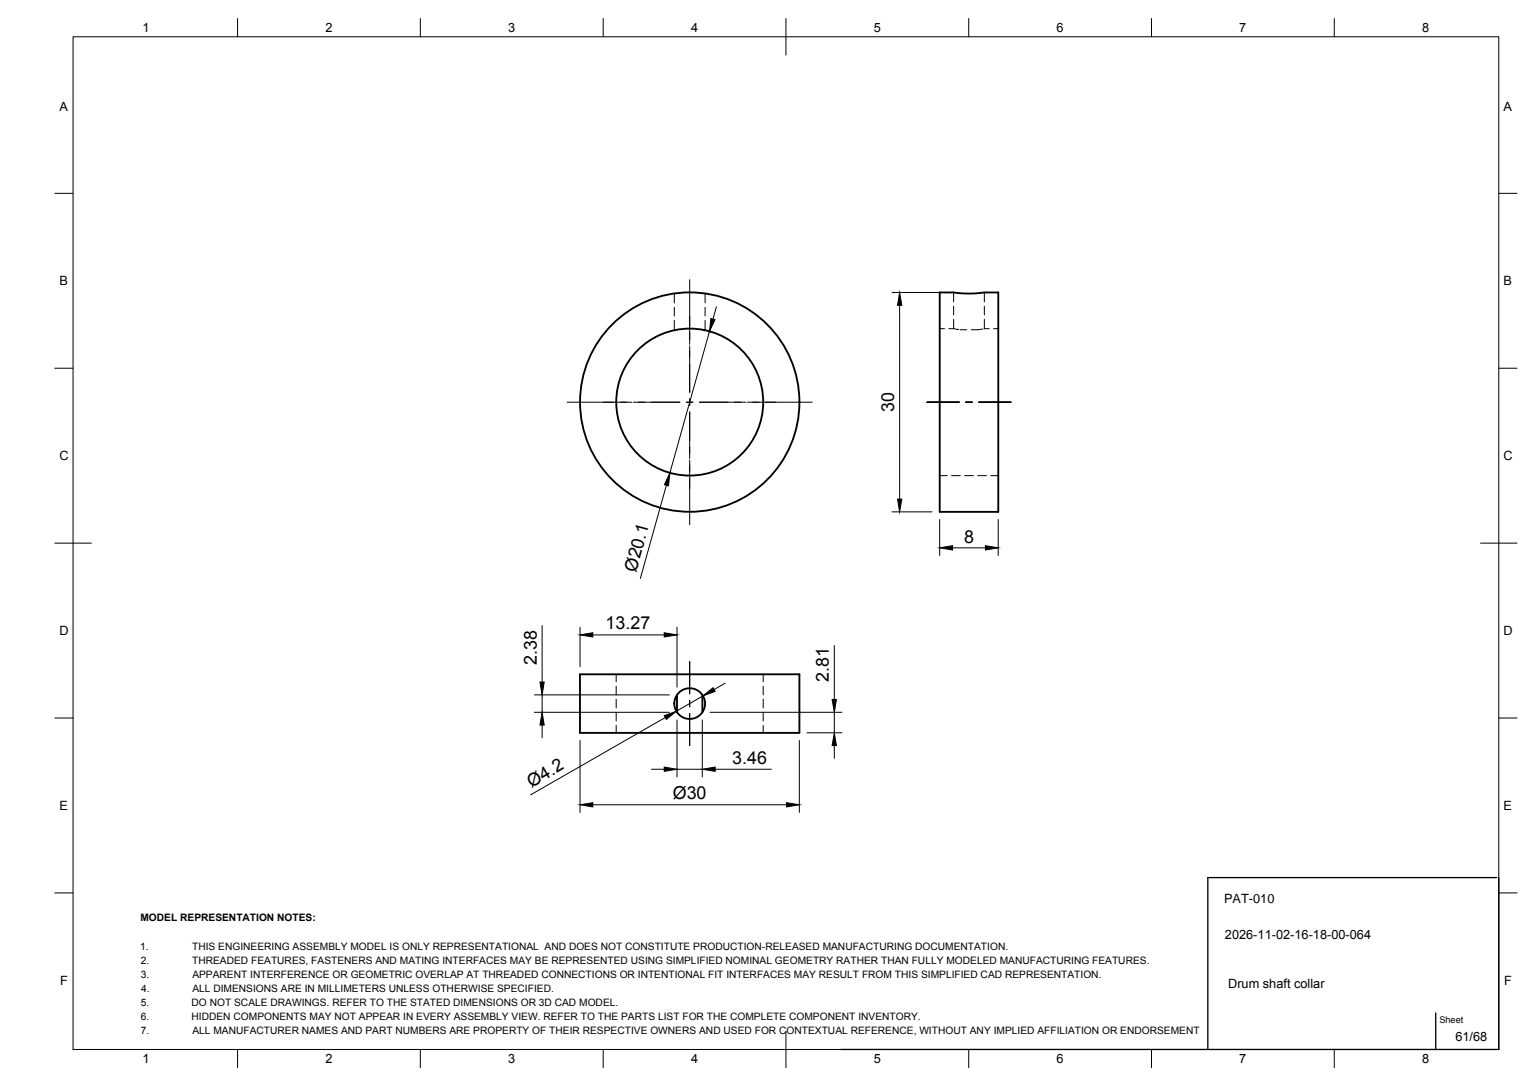
ISO-10303-21;
HEADER;
/* Generated by software containing ST-Developer
 * from STEP Tools, Inc. (www.steptools.com) 
 */

FILE_DESCRIPTION(
/* description */ ('Belt conveyor head drive unit'),
/* implementation_level */ '2;1');

FILE_NAME(
/* name */ 'Drum shaft collar.step',
/* time_stamp */ '2026-10-28T03:26:19-07:00',
/* author */ (''),
/* organization */ (''),
/* preprocessor_version */ 'ST-DEVELOPER v20.2',
/* originating_system */ 'Autodesk Translation Framework v15.17.0.0',
/* authorisation */ '');

FILE_SCHEMA (('AUTOMOTIVE_DESIGN { 1 0 10303 214 3 1 1 }'));
ENDSEC;

DATA;
#10=MECHANICAL_DESIGN_GEOMETRIC_PRESENTATION_REPRESENTATION('',(#922),#27069);
#607=B_SPLINE_CURVE_WITH_KNOTS('',3,(#25420,#25421,#25422,#25423,#25424,
#25425,#25426,#25427,#25428,#25429,#25430,#25431,#25432,#25433),
 .UNSPECIFIED.,.F.,.F.,(4,2,2,2,2,2,4),(0.756005737987021,0.793568827564646,
0.872922520054201,0.952276212543756,1.03162990503331,1.11098359752286,1.14854668710049),
 .UNSPECIFIED.);
#608=B_SPLINE_CURVE_WITH_KNOTS('',3,(#25439,#25440,#25441,#25442,#25443,
#25444,#25445,#25446,#25447,#25448,#25449,#25450,#25451,#25452,#25453,#25454,
#25455,#25456),.UNSPECIFIED.,.F.,.F.,(4,2,2,2,2,2,2,2,4),(0.,0.0792165807733631,
0.158433161546726,0.23764869707457,0.316864232602414,0.396079768130258,
0.475295303658102,0.554511884431466,0.633728465204829),.UNSPECIFIED.);
#609=B_SPLINE_CURVE_WITH_KNOTS('',3,(#25457,#25458,#25459,#25460,#25461,
#25462,#25463,#25464,#25465,#25466,#25467,#25468,#25469,#25470,#25471,#25472,
#25473,#25474),.UNSPECIFIED.,.F.,.F.,(4,2,2,2,2,2,2,2,4),(0.633728465204829,
0.712945045978192,0.792161626751554,0.871377162279399,0.950592697807243,
1.02980823333509,1.10902376886293,1.18824034963629,1.26745693040966),
 .UNSPECIFIED.);
#610=B_SPLINE_CURVE_WITH_KNOTS('',3,(#25477,#25478,#25479,#25480,#25481,
#25482,#25483,#25484,#25485,#25486,#25487,#25488,#25489,#25490),
 .UNSPECIFIED.,.F.,.F.,(4,2,2,2,2,2,4),(0.121154929624517,0.158718019202143,
0.238071711691697,0.317425404181252,0.396779096670806,0.476132789160361,
0.513695878737986),.UNSPECIFIED.);
#768=SHAPE_REPRESENTATION_RELATIONSHIP('SRR','None',#27417,#837);
#837=ADVANCED_BREP_SHAPE_REPRESENTATION('',(#1003),#27059);
#922=STYLED_ITEM('',(#27797),#1003);
#1003=MANIFOLD_SOLID_BREP('Body1',#13791);
#1242=FACE_BOUND('',#3305,.T.);
#1243=FACE_BOUND('',#3307,.T.);
#1244=FACE_BOUND('',#3309,.T.);
#1245=FACE_BOUND('',#3311,.T.);
#1586=PLANE('',#15930);
#1587=PLANE('',#15935);
#1588=PLANE('',#15942);
#1589=PLANE('',#15943);
#2271=FACE_OUTER_BOUND('',#3301,.T.);
#2272=FACE_OUTER_BOUND('',#3302,.T.);
#2273=FACE_OUTER_BOUND('',#3303,.T.);
#2274=FACE_OUTER_BOUND('',#3304,.T.);
#2275=FACE_OUTER_BOUND('',#3306,.T.);
#2276=FACE_OUTER_BOUND('',#3308,.T.);
#2277=FACE_OUTER_BOUND('',#3310,.T.);
#3301=EDGE_LOOP('',(#11694,#11695));
#3302=EDGE_LOOP('',(#11696,#11697,#11698,#11699,#11700,#11701,#11702,#11703,
#11704));
#3303=EDGE_LOOP('',(#11705,#11706,#11707));
#3304=EDGE_LOOP('',(#11708,#11709,#11710,#11711));
#3305=EDGE_LOOP('',(#11712,#11713,#11714,#11715));
#3306=EDGE_LOOP('',(#11716,#11717,#11718,#11719));
#3307=EDGE_LOOP('',(#11720,#11721));
#3308=EDGE_LOOP('',(#11722));
#3309=EDGE_LOOP('',(#11723));
#3310=EDGE_LOOP('',(#11724));
#3311=EDGE_LOOP('',(#11725));
#4129=LINE('',#25416,#4921);
#4130=LINE('',#25437,#4922);
#4131=LINE('',#25492,#4923);
#4132=LINE('',#25497,#4924);
#4133=LINE('',#25503,#4925);
#4921=VECTOR('',#19803,1.);
#4922=VECTOR('',#19810,0.21);
#4923=VECTOR('',#19815,1.);
#4924=VECTOR('',#19820,1.005);
#4925=VECTOR('',#19827,1.5);
#5733=CIRCLE('',#15931,0.21);
#5734=CIRCLE('',#15933,0.21);
#5735=CIRCLE('',#15934,0.21);
#5736=CIRCLE('',#15937,1.005);
#5737=CIRCLE('',#15938,1.005);
#5738=CIRCLE('',#15940,1.5);
#5739=CIRCLE('',#15941,1.5);
#6889=VERTEX_POINT('',#25414);
#6890=VERTEX_POINT('',#25415);
#6891=VERTEX_POINT('',#25419);
#6892=VERTEX_POINT('',#25434);
#6893=VERTEX_POINT('',#25436);
#6894=VERTEX_POINT('',#25438);
#6895=VERTEX_POINT('',#25475);
#6896=VERTEX_POINT('',#25494);
#6897=VERTEX_POINT('',#25496);
#6898=VERTEX_POINT('',#25500);
#6899=VERTEX_POINT('',#25502);
#8539=EDGE_CURVE('',#6889,#6890,#4129,.T.);
#8540=EDGE_CURVE('',#6889,#6890,#5733,.T.);
#8541=EDGE_CURVE('',#6891,#6889,#607,.T.);
#8542=EDGE_CURVE('',#6892,#6891,#5734,.T.);
#8543=EDGE_CURVE('',#6892,#6893,#4130,.T.);
#8544=EDGE_CURVE('',#6894,#6893,#608,.T.);
#8545=EDGE_CURVE('',#6893,#6894,#609,.T.);
#8546=EDGE_CURVE('',#6895,#6892,#5735,.T.);
#8547=EDGE_CURVE('',#6890,#6895,#610,.T.);
#8548=EDGE_CURVE('',#6895,#6891,#4131,.T.);
#8549=EDGE_CURVE('',#6896,#6896,#5736,.T.);
#8550=EDGE_CURVE('',#6896,#6897,#4132,.T.);
#8551=EDGE_CURVE('',#6897,#6897,#5737,.T.);
#8552=EDGE_CURVE('',#6898,#6898,#5738,.T.);
#8553=EDGE_CURVE('',#6898,#6899,#4133,.T.);
#8554=EDGE_CURVE('',#6899,#6899,#5739,.T.);
#11694=ORIENTED_EDGE('',*,*,#8539,.F.);
#11695=ORIENTED_EDGE('',*,*,#8540,.T.);
#11696=ORIENTED_EDGE('',*,*,#8541,.F.);
#11697=ORIENTED_EDGE('',*,*,#8542,.F.);
#11698=ORIENTED_EDGE('',*,*,#8543,.T.);
#11699=ORIENTED_EDGE('',*,*,#8544,.F.);
#11700=ORIENTED_EDGE('',*,*,#8545,.F.);
#11701=ORIENTED_EDGE('',*,*,#8543,.F.);
#11702=ORIENTED_EDGE('',*,*,#8546,.F.);
#11703=ORIENTED_EDGE('',*,*,#8547,.F.);
#11704=ORIENTED_EDGE('',*,*,#8540,.F.);
#11705=ORIENTED_EDGE('',*,*,#8548,.F.);
#11706=ORIENTED_EDGE('',*,*,#8546,.T.);
#11707=ORIENTED_EDGE('',*,*,#8542,.T.);
#11708=ORIENTED_EDGE('',*,*,#8549,.F.);
#11709=ORIENTED_EDGE('',*,*,#8550,.T.);
#11710=ORIENTED_EDGE('',*,*,#8551,.T.);
#11711=ORIENTED_EDGE('',*,*,#8550,.F.);
#11712=ORIENTED_EDGE('',*,*,#8547,.T.);
#11713=ORIENTED_EDGE('',*,*,#8548,.T.);
#11714=ORIENTED_EDGE('',*,*,#8541,.T.);
#11715=ORIENTED_EDGE('',*,*,#8539,.T.);
#11716=ORIENTED_EDGE('',*,*,#8552,.F.);
#11717=ORIENTED_EDGE('',*,*,#8553,.T.);
#11718=ORIENTED_EDGE('',*,*,#8554,.T.);
#11719=ORIENTED_EDGE('',*,*,#8553,.F.);
#11720=ORIENTED_EDGE('',*,*,#8544,.T.);
#11721=ORIENTED_EDGE('',*,*,#8545,.T.);
#11722=ORIENTED_EDGE('',*,*,#8552,.T.);
#11723=ORIENTED_EDGE('',*,*,#8549,.T.);
#11724=ORIENTED_EDGE('',*,*,#8554,.F.);
#11725=ORIENTED_EDGE('',*,*,#8551,.F.);
#12803=CYLINDRICAL_SURFACE('',#15932,0.21);
#12804=CYLINDRICAL_SURFACE('',#15936,1.005);
#12805=CYLINDRICAL_SURFACE('',#15939,1.5);
#13550=ADVANCED_FACE('',(#2271),#1586,.T.);
#13551=ADVANCED_FACE('',(#2272),#12803,.F.);
#13552=ADVANCED_FACE('',(#2273),#1587,.T.);
#13553=ADVANCED_FACE('',(#2274,#1242),#12804,.F.);
#13554=ADVANCED_FACE('',(#2275,#1243),#12805,.T.);
#13555=ADVANCED_FACE('',(#2276,#1244),#1588,.T.);
#13556=ADVANCED_FACE('',(#2277,#1245),#1589,.F.);
#13791=CLOSED_SHELL('',(#13550,#13551,#13552,#13553,#13554,#13555,#13556));
#15929=AXIS2_PLACEMENT_3D('',#25412,#19799,#19800);
#15930=AXIS2_PLACEMENT_3D('',#25413,#19801,#19802);
#15931=AXIS2_PLACEMENT_3D('',#25417,#19804,#19805);
#15932=AXIS2_PLACEMENT_3D('',#25418,#19806,#19807);
#15933=AXIS2_PLACEMENT_3D('',#25435,#19808,#19809);
#15934=AXIS2_PLACEMENT_3D('',#25476,#19811,#19812);
#15935=AXIS2_PLACEMENT_3D('',#25491,#19813,#19814);
#15936=AXIS2_PLACEMENT_3D('',#25493,#19816,#19817);
#15937=AXIS2_PLACEMENT_3D('',#25495,#19818,#19819);
#15938=AXIS2_PLACEMENT_3D('',#25498,#19821,#19822);
#15939=AXIS2_PLACEMENT_3D('',#25499,#19823,#19824);
#15940=AXIS2_PLACEMENT_3D('',#25501,#19825,#19826);
#15941=AXIS2_PLACEMENT_3D('',#25504,#19828,#19829);
#15942=AXIS2_PLACEMENT_3D('',#25505,#19830,#19831);
#15943=AXIS2_PLACEMENT_3D('',#25506,#19832,#19833);
#19799=DIRECTION('axis',(0.,0.,1.));
#19800=DIRECTION('refdir',(1.,0.,0.));
#19801=DIRECTION('center_axis',(0.,0.,1.));
#19802=DIRECTION('ref_axis',(1.,0.,0.));
#19803=DIRECTION('',(0.,1.,0.));
#19804=DIRECTION('center_axis',(0.,0.,1.));
#19805=DIRECTION('ref_axis',(1.,0.,0.));
#19806=DIRECTION('center_axis',(0.,0.,1.));
#19807=DIRECTION('ref_axis',(1.,0.,0.));
#19808=DIRECTION('center_axis',(0.,0.,1.));
#19809=DIRECTION('ref_axis',(1.,0.,0.));
#19810=DIRECTION('',(0.,0.,1.));
#19811=DIRECTION('center_axis',(0.,0.,1.));
#19812=DIRECTION('ref_axis',(1.,0.,0.));
#19813=DIRECTION('center_axis',(0.,0.,1.));
#19814=DIRECTION('ref_axis',(1.,0.,0.));
#19815=DIRECTION('',(0.,-1.,0.));
#19816=DIRECTION('center_axis',(0.,1.,0.));
#19817=DIRECTION('ref_axis',(1.,0.,0.));
#19818=DIRECTION('center_axis',(0.,-1.,0.));
#19819=DIRECTION('ref_axis',(1.,0.,0.));
#19820=DIRECTION('',(0.,-1.,0.));
#19821=DIRECTION('center_axis',(0.,-1.,0.));
#19822=DIRECTION('ref_axis',(1.,0.,0.));
#19823=DIRECTION('center_axis',(0.,1.,0.));
#19824=DIRECTION('ref_axis',(1.,0.,0.));
#19825=DIRECTION('center_axis',(0.,1.,0.));
#19826=DIRECTION('ref_axis',(1.,0.,0.));
#19827=DIRECTION('',(0.,-1.,0.));
#19828=DIRECTION('center_axis',(0.,1.,0.));
#19829=DIRECTION('ref_axis',(1.,0.,0.));
#19830=DIRECTION('center_axis',(0.,1.,0.));
#19831=DIRECTION('ref_axis',(1.,0.,0.));
#19832=DIRECTION('center_axis',(0.,1.,0.));
#19833=DIRECTION('ref_axis',(1.,0.,0.));
#25412=CARTESIAN_POINT('',(0.,0.,0.));
#25413=CARTESIAN_POINT('Origin',(6.97091003018116,2.75,7.99));
#25414=CARTESIAN_POINT('',(7.14389846910121,2.63094119100208,7.99));
#25415=CARTESIAN_POINT('',(7.14389846910121,2.86905880899792,7.99));
#25416=CARTESIAN_POINT('',(7.14389846910121,2.35,7.99));
#25417=CARTESIAN_POINT('Origin',(6.97091003018116,2.75,7.99));
#25418=CARTESIAN_POINT('Origin',(6.97091003018116,2.75,7.99));
#25419=CARTESIAN_POINT('',(6.7979215912611,2.63094119100208,7.99));
#25420=CARTESIAN_POINT('Ctrl Pts',(6.7979215912611,2.63094119100208,7.99));
#25421=CARTESIAN_POINT('Ctrl Pts',(6.80531516486984,2.62019857760471,7.99129192197638));
#25422=CARTESIAN_POINT('Ctrl Pts',(6.81361289145555,2.61031229062726,7.99265394943905));
#25423=CARTESIAN_POINT('Ctrl Pts',(6.84101795633608,2.58290722574673,7.9967480843909));
#25424=CARTESIAN_POINT('Ctrl Pts',(6.86457986242187,2.56675794366705,7.99969589327638));
#25425=CARTESIAN_POINT('Ctrl Pts',(6.91629712554874,2.54530220603509,8.00385029472357));
#25426=CARTESIAN_POINT('Ctrl Pts',(6.9444587993513,2.54,8.005));
#25427=CARTESIAN_POINT('Ctrl Pts',(6.99736126101101,2.54,8.005));
#25428=CARTESIAN_POINT('Ctrl Pts',(7.02552293481357,2.54530220603509,8.00385029472357));
#25429=CARTESIAN_POINT('Ctrl Pts',(7.07724019794044,2.56675794366705,7.99969589327638));
#25430=CARTESIAN_POINT('Ctrl Pts',(7.10080210402623,2.58290722574673,7.9967480843909));
#25431=CARTESIAN_POINT('Ctrl Pts',(7.12820716890676,2.61031229062726,7.99265394943905));
#25432=CARTESIAN_POINT('Ctrl Pts',(7.13650489549247,2.62019857760471,7.99129192197638));
#25433=CARTESIAN_POINT('Ctrl Pts',(7.14389846910121,2.63094119100208,7.99));
#25434=CARTESIAN_POINT('',(6.76091003018116,2.75,7.99));
#25435=CARTESIAN_POINT('Origin',(6.97091003018116,2.75,7.99));
#25436=CARTESIAN_POINT('',(6.76091003018116,2.75,8.48522725533839));
#25437=CARTESIAN_POINT('',(6.76091003018116,2.75,7.99));
#25438=CARTESIAN_POINT('',(7.18091003018116,2.75,8.48522725533839));
#25439=CARTESIAN_POINT('Ctrl Pts',(7.18091003018116,2.75,8.48522725533839));
#25440=CARTESIAN_POINT('Ctrl Pts',(7.18091003018116,2.72359447307555,8.48522725533839));
#25441=CARTESIAN_POINT('Ctrl Pts',(7.17562576745075,2.69545292590929,8.48600415954412));
#25442=CARTESIAN_POINT('Ctrl Pts',(7.15418379321749,2.64372373109487,8.48880073282317));
#25443=CARTESIAN_POINT('Ctrl Pts',(7.13802795415155,2.62013307587204,8.49077897157582));
#25444=CARTESIAN_POINT('Ctrl Pts',(7.10077720006852,2.58288232178902,8.49448481141327));
#25445=CARTESIAN_POINT('Ctrl Pts',(7.07718643848692,2.56672628999865,8.49645455657129));
#25446=CARTESIAN_POINT('Ctrl Pts',(7.02545688158706,2.54528417517378,8.49923165515645));
#25447=CARTESIAN_POINT('Ctrl Pts',(6.99731520869044,2.54,8.5));
#25448=CARTESIAN_POINT('Ctrl Pts',(6.94450485167187,2.54,8.5));
#25449=CARTESIAN_POINT('Ctrl Pts',(6.91636317877526,2.54528417517378,8.49923165515645));
#25450=CARTESIAN_POINT('Ctrl Pts',(6.86463362187539,2.56672628999865,8.49645455657129));
#25451=CARTESIAN_POINT('Ctrl Pts',(6.84104286029379,2.58288232178902,8.49448481141327));
#25452=CARTESIAN_POINT('Ctrl Pts',(6.80379210621076,2.62013307587204,8.49077897157582));
#25453=CARTESIAN_POINT('Ctrl Pts',(6.78763626714482,2.64372373109487,8.48880073282317));
#25454=CARTESIAN_POINT('Ctrl Pts',(6.76619429291156,2.69545292590929,8.48600415954412));
#25455=CARTESIAN_POINT('Ctrl Pts',(6.76091003018116,2.72359447307555,8.48522725533839));
#25456=CARTESIAN_POINT('Ctrl Pts',(6.76091003018116,2.75,8.48522725533839));
#25457=CARTESIAN_POINT('Ctrl Pts',(6.76091003018116,2.75,8.48522725533839));
#25458=CARTESIAN_POINT('Ctrl Pts',(6.76091003018116,2.77640552692445,8.48522725533839));
#25459=CARTESIAN_POINT('Ctrl Pts',(6.76619429291156,2.80454707409071,8.48600415954412));
#25460=CARTESIAN_POINT('Ctrl Pts',(6.78763626714482,2.85627626890513,8.48880073282317));
#25461=CARTESIAN_POINT('Ctrl Pts',(6.80379210621076,2.87986692412796,8.49077897157582));
#25462=CARTESIAN_POINT('Ctrl Pts',(6.84104286029379,2.91711767821098,8.49448481141327));
#25463=CARTESIAN_POINT('Ctrl Pts',(6.86463362187539,2.93327371000135,8.49645455657129));
#25464=CARTESIAN_POINT('Ctrl Pts',(6.91636317877526,2.95471582482622,8.49923165515645));
#25465=CARTESIAN_POINT('Ctrl Pts',(6.94450485167187,2.96,8.5));
#25466=CARTESIAN_POINT('Ctrl Pts',(6.99731520869044,2.96,8.5));
#25467=CARTESIAN_POINT('Ctrl Pts',(7.02545688158706,2.95471582482622,8.49923165515645));
#25468=CARTESIAN_POINT('Ctrl Pts',(7.07718643848692,2.93327371000135,8.49645455657129));
#25469=CARTESIAN_POINT('Ctrl Pts',(7.10077720006852,2.91711767821098,8.49448481141327));
#25470=CARTESIAN_POINT('Ctrl Pts',(7.13802795415155,2.87986692412796,8.49077897157582));
#25471=CARTESIAN_POINT('Ctrl Pts',(7.15418379321749,2.85627626890513,8.48880073282317));
#25472=CARTESIAN_POINT('Ctrl Pts',(7.17562576745075,2.80454707409071,8.48600415954412));
#25473=CARTESIAN_POINT('Ctrl Pts',(7.18091003018116,2.77640552692445,8.48522725533839));
#25474=CARTESIAN_POINT('Ctrl Pts',(7.18091003018116,2.75,8.48522725533839));
#25475=CARTESIAN_POINT('',(6.7979215912611,2.86905880899792,7.99));
#25476=CARTESIAN_POINT('Origin',(6.97091003018116,2.75,7.99));
#25477=CARTESIAN_POINT('Ctrl Pts',(7.14389846910121,2.86905880899792,7.99));
#25478=CARTESIAN_POINT('Ctrl Pts',(7.13650489549247,2.87980142239529,7.99129192197638));
#25479=CARTESIAN_POINT('Ctrl Pts',(7.12820716890676,2.88968770937274,7.99265394943905));
#25480=CARTESIAN_POINT('Ctrl Pts',(7.10080210402623,2.91709277425327,7.9967480843909));
#25481=CARTESIAN_POINT('Ctrl Pts',(7.07724019794044,2.93324205633295,7.99969589327638));
#25482=CARTESIAN_POINT('Ctrl Pts',(7.02552293481357,2.95469779396491,8.00385029472357));
#25483=CARTESIAN_POINT('Ctrl Pts',(6.99736126101101,2.96,8.005));
#25484=CARTESIAN_POINT('Ctrl Pts',(6.9444587993513,2.96,8.005));
#25485=CARTESIAN_POINT('Ctrl Pts',(6.91629712554875,2.95469779396491,8.00385029472357));
#25486=CARTESIAN_POINT('Ctrl Pts',(6.86457986242187,2.93324205633295,7.99969589327638));
#25487=CARTESIAN_POINT('Ctrl Pts',(6.84101795633608,2.91709277425327,7.9967480843909));
#25488=CARTESIAN_POINT('Ctrl Pts',(6.81361289145555,2.88968770937274,7.99265394943905));
#25489=CARTESIAN_POINT('Ctrl Pts',(6.80531516486984,2.87980142239529,7.99129192197638));
#25490=CARTESIAN_POINT('Ctrl Pts',(6.7979215912611,2.86905880899792,7.99));
#25491=CARTESIAN_POINT('Origin',(6.97091003018116,2.75,7.99));
#25492=CARTESIAN_POINT('',(6.7979215912611,2.35,7.99));
#25493=CARTESIAN_POINT('Origin',(6.97091003018116,2.35,7.));
#25494=CARTESIAN_POINT('',(5.96591003018116,3.15,7.));
#25495=CARTESIAN_POINT('Origin',(6.97091003018116,3.15,7.));
#25496=CARTESIAN_POINT('',(5.96591003018116,2.35,7.));
#25497=CARTESIAN_POINT('',(5.96591003018116,2.35,7.));
#25498=CARTESIAN_POINT('Origin',(6.97091003018116,2.35,7.));
#25499=CARTESIAN_POINT('Origin',(6.97091003018116,2.35,7.));
#25500=CARTESIAN_POINT('',(5.47091003018116,3.15,7.));
#25501=CARTESIAN_POINT('Origin',(6.97091003018116,3.15,7.));
#25502=CARTESIAN_POINT('',(5.47091003018116,2.35,7.));
#25503=CARTESIAN_POINT('',(5.47091003018116,2.35,7.));
#25504=CARTESIAN_POINT('Origin',(6.97091003018116,2.35,7.));
#25505=CARTESIAN_POINT('Origin',(6.97091003018116,3.15,7.));
#25506=CARTESIAN_POINT('Origin',(6.97091003018116,2.35,7.));
#26982=UNCERTAINTY_MEASURE_WITH_UNIT(LENGTH_MEASURE(0.001),#27070,
'DISTANCE_ACCURACY_VALUE',
'Maximum model space distance between geometric entities at asserted c
onnectivities');
#26992=UNCERTAINTY_MEASURE_WITH_UNIT(LENGTH_MEASURE(0.001),#27070,
'DISTANCE_ACCURACY_VALUE',
'Maximum model space distance between geometric entities at asserted c
onnectivities');
#27059=(
GEOMETRIC_REPRESENTATION_CONTEXT(3)
GLOBAL_UNCERTAINTY_ASSIGNED_CONTEXT((#26982))
GLOBAL_UNIT_ASSIGNED_CONTEXT((#27070,#27072,#27073))
REPRESENTATION_CONTEXT('','3D')
);
#27069=(
GEOMETRIC_REPRESENTATION_CONTEXT(3)
GLOBAL_UNCERTAINTY_ASSIGNED_CONTEXT((#26992))
GLOBAL_UNIT_ASSIGNED_CONTEXT((#27070,#27072,#27073))
REPRESENTATION_CONTEXT('','3D')
);
#27070=(
LENGTH_UNIT()
NAMED_UNIT(*)
SI_UNIT(.CENTI.,.METRE.)
);
#27072=(
NAMED_UNIT(*)
PLANE_ANGLE_UNIT()
SI_UNIT($,.RADIAN.)
);
#27073=(
NAMED_UNIT(*)
SI_UNIT($,.STERADIAN.)
SOLID_ANGLE_UNIT()
);
#27140=SHAPE_DEFINITION_REPRESENTATION(#27228,#27417);
#27228=PRODUCT_DEFINITION_SHAPE('',$,#27494);
#27417=SHAPE_REPRESENTATION('',(#15929),#27059);
#27427=PRODUCT_DEFINITION_CONTEXT('part definition',#27657,'design');
#27494=PRODUCT_DEFINITION('Drum shaft collar','Drum shaft collar',#27570,
#27427);
#27570=PRODUCT_DEFINITION_FORMATION('',$,#27725);
#27657=APPLICATION_CONTEXT(
'Core Data for Automotive Mechanical Design Process');
#27658=PRODUCT_CONTEXT('part definition',#27657,'mechanical');
#27725=PRODUCT('Drum shaft collar','Drum shaft collar',
'Drum shaft collar',(#27658));
#27791=COLOUR_RGB('Grey',0.48,0.52,0.57);
#27792=FILL_AREA_STYLE_COLOUR('',#27791);
#27793=FILL_AREA_STYLE('',(#27792));
#27794=SURFACE_STYLE_FILL_AREA(#27793);
#27795=SURFACE_SIDE_STYLE('',(#27794));
#27796=SURFACE_STYLE_USAGE(.BOTH.,#27795);
#27797=PRESENTATION_STYLE_ASSIGNMENT((#27796));
ENDSEC;
END-ISO-10303-21;
